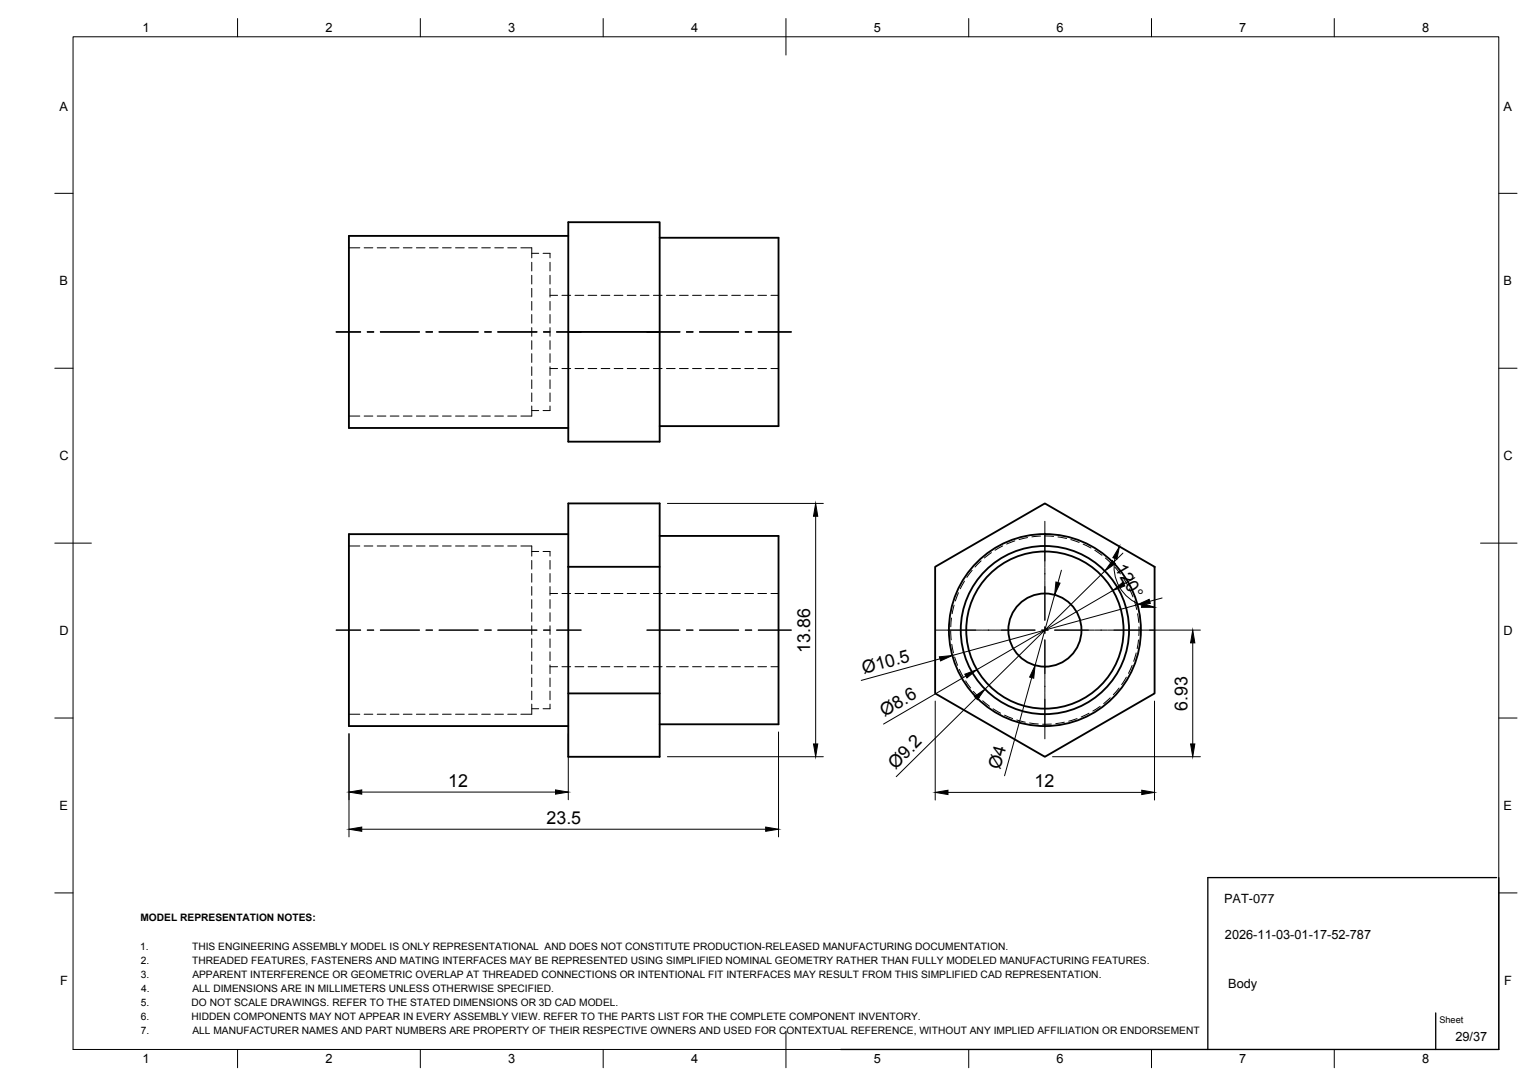
ISO-10303-21;
HEADER;
/* Generated by software containing ST-Developer
 * from STEP Tools, Inc. (www.steptools.com) 
 */

FILE_DESCRIPTION(
/* description */ ('Pallet stop with pneumatic fitting'),
/* implementation_level */ '2;1');

FILE_NAME(
/* name */ 'Body.step',
/* time_stamp */ '2026-10-27T10:51:41-07:00',
/* author */ (''),
/* organization */ (''),
/* preprocessor_version */ 'ST-DEVELOPER v20.2',
/* originating_system */ 'Autodesk Translation Framework v15.17.0.0',
/* authorisation */ '');

FILE_SCHEMA (('AUTOMOTIVE_DESIGN { 1 0 10303 214 3 1 1 }'));
ENDSEC;

DATA;
#10=MECHANICAL_DESIGN_GEOMETRIC_PRESENTATION_REPRESENTATION('',(#378),#10265);
#314=SHAPE_REPRESENTATION_RELATIONSHIP('SRR','None',#10429,#346);
#346=ADVANCED_BREP_SHAPE_REPRESENTATION('',(#409),#10253);
#378=STYLED_ITEM('',(#10634),#409);
#409=MANIFOLD_SOLID_BREP('Body1',#5067);
#516=FACE_BOUND('',#1349,.T.);
#517=FACE_BOUND('',#1351,.T.);
#518=FACE_BOUND('',#1353,.T.);
#519=FACE_BOUND('',#1361,.T.);
#520=FACE_BOUND('',#1364,.T.);
#521=FACE_BOUND('',#1368,.T.);
#660=PLANE('',#5834);
#661=PLANE('',#5836);
#662=PLANE('',#5838);
#663=PLANE('',#5840);
#664=PLANE('',#5841);
#665=PLANE('',#5842);
#666=PLANE('',#5843);
#667=PLANE('',#5844);
#668=PLANE('',#5845);
#669=PLANE('',#5846);
#670=PLANE('',#5850);
#671=PLANE('',#5855);
#936=FACE_OUTER_BOUND('',#1347,.T.);
#937=FACE_OUTER_BOUND('',#1348,.T.);
#938=FACE_OUTER_BOUND('',#1350,.T.);
#939=FACE_OUTER_BOUND('',#1352,.T.);
#940=FACE_OUTER_BOUND('',#1354,.T.);
#941=FACE_OUTER_BOUND('',#1355,.T.);
#942=FACE_OUTER_BOUND('',#1356,.T.);
#943=FACE_OUTER_BOUND('',#1357,.T.);
#944=FACE_OUTER_BOUND('',#1358,.T.);
#945=FACE_OUTER_BOUND('',#1359,.T.);
#946=FACE_OUTER_BOUND('',#1360,.T.);
#947=FACE_OUTER_BOUND('',#1362,.T.);
#948=FACE_OUTER_BOUND('',#1363,.T.);
#949=FACE_OUTER_BOUND('',#1365,.T.);
#950=FACE_OUTER_BOUND('',#1366,.T.);
#951=FACE_OUTER_BOUND('',#1367,.T.);
#952=FACE_OUTER_BOUND('',#1369,.T.);
#1347=EDGE_LOOP('',(#4160,#4161,#4162,#4163));
#1348=EDGE_LOOP('',(#4164));
#1349=EDGE_LOOP('',(#4165));
#1350=EDGE_LOOP('',(#4166,#4167,#4168,#4169,#4170,#4171));
#1351=EDGE_LOOP('',(#4172));
#1352=EDGE_LOOP('',(#4173,#4174,#4175,#4176,#4177,#4178));
#1353=EDGE_LOOP('',(#4179));
#1354=EDGE_LOOP('',(#4180,#4181,#4182,#4183));
#1355=EDGE_LOOP('',(#4184,#4185,#4186,#4187));
#1356=EDGE_LOOP('',(#4188,#4189,#4190,#4191));
#1357=EDGE_LOOP('',(#4192,#4193,#4194,#4195));
#1358=EDGE_LOOP('',(#4196,#4197,#4198,#4199));
#1359=EDGE_LOOP('',(#4200,#4201,#4202,#4203));
#1360=EDGE_LOOP('',(#4204));
#1361=EDGE_LOOP('',(#4205));
#1362=EDGE_LOOP('',(#4206,#4207,#4208,#4209));
#1363=EDGE_LOOP('',(#4210));
#1364=EDGE_LOOP('',(#4211));
#1365=EDGE_LOOP('',(#4212,#4213,#4214,#4215));
#1366=EDGE_LOOP('',(#4216,#4217,#4218,#4219));
#1367=EDGE_LOOP('',(#4220));
#1368=EDGE_LOOP('',(#4221));
#1369=EDGE_LOOP('',(#4222,#4223,#4224,#4225));
#1686=LINE('',#9545,#2021);
#1687=LINE('',#9553,#2022);
#1688=LINE('',#9555,#2023);
#1689=LINE('',#9557,#2024);
#1690=LINE('',#9559,#2025);
#1691=LINE('',#9561,#2026);
#1692=LINE('',#9562,#2027);
#1693=LINE('',#9568,#2028);
#1694=LINE('',#9570,#2029);
#1695=LINE('',#9572,#2030);
#1696=LINE('',#9574,#2031);
#1697=LINE('',#9576,#2032);
#1698=LINE('',#9577,#2033);
#1699=LINE('',#9581,#2034);
#1700=LINE('',#9582,#2035);
#1701=LINE('',#9584,#2036);
#1702=LINE('',#9586,#2037);
#1703=LINE('',#9588,#2038);
#1704=LINE('',#9590,#2039);
#1705=LINE('',#9597,#2040);
#1706=LINE('',#9603,#2041);
#1707=LINE('',#9607,#2042);
#1708=LINE('',#9612,#2043);
#2021=VECTOR('',#7087,0.43);
#2022=VECTOR('',#7096,1.);
#2023=VECTOR('',#7097,1.);
#2024=VECTOR('',#7098,1.);
#2025=VECTOR('',#7099,1.);
#2026=VECTOR('',#7100,1.);
#2027=VECTOR('',#7101,1.);
#2028=VECTOR('',#7106,1.);
#2029=VECTOR('',#7107,1.);
#2030=VECTOR('',#7108,1.);
#2031=VECTOR('',#7109,1.);
#2032=VECTOR('',#7110,1.);
#2033=VECTOR('',#7111,1.);
#2034=VECTOR('',#7116,1.);
#2035=VECTOR('',#7117,1.);
#2036=VECTOR('',#7120,1.);
#2037=VECTOR('',#7123,1.);
#2038=VECTOR('',#7126,1.);
#2039=VECTOR('',#7129,1.);
#2040=VECTOR('',#7138,0.46);
#2041=VECTOR('',#7147,0.525);
#2042=VECTOR('',#7152,0.515);
#2043=VECTOR('',#7159,0.2);
#2332=CIRCLE('',#5832,0.43);
#2333=CIRCLE('',#5833,0.43);
#2334=CIRCLE('',#5835,0.2);
#2335=CIRCLE('',#5837,0.525);
#2336=CIRCLE('',#5839,0.515);
#2337=CIRCLE('',#5847,0.46);
#2338=CIRCLE('',#5849,0.46);
#2339=CIRCLE('',#5851,0.525);
#2340=CIRCLE('',#5854,0.515);
#2341=CIRCLE('',#5856,0.2);
#2654=VERTEX_POINT('',#9542);
#2655=VERTEX_POINT('',#9544);
#2656=VERTEX_POINT('',#9548);
#2657=VERTEX_POINT('',#9551);
#2658=VERTEX_POINT('',#9552);
#2659=VERTEX_POINT('',#9554);
#2660=VERTEX_POINT('',#9556);
#2661=VERTEX_POINT('',#9558);
#2662=VERTEX_POINT('',#9560);
#2663=VERTEX_POINT('',#9563);
#2664=VERTEX_POINT('',#9566);
#2665=VERTEX_POINT('',#9567);
#2666=VERTEX_POINT('',#9569);
#2667=VERTEX_POINT('',#9571);
#2668=VERTEX_POINT('',#9573);
#2669=VERTEX_POINT('',#9575);
#2670=VERTEX_POINT('',#9578);
#2671=VERTEX_POINT('',#9593);
#2672=VERTEX_POINT('',#9596);
#2673=VERTEX_POINT('',#9600);
#2674=VERTEX_POINT('',#9605);
#2675=VERTEX_POINT('',#9609);
#3179=EDGE_CURVE('',#2654,#2654,#2332,.T.);
#3180=EDGE_CURVE('',#2654,#2655,#1686,.T.);
#3181=EDGE_CURVE('',#2655,#2655,#2333,.T.);
#3182=EDGE_CURVE('',#2656,#2656,#2334,.T.);
#3183=EDGE_CURVE('',#2657,#2658,#1687,.T.);
#3184=EDGE_CURVE('',#2658,#2659,#1688,.T.);
#3185=EDGE_CURVE('',#2659,#2660,#1689,.T.);
#3186=EDGE_CURVE('',#2660,#2661,#1690,.T.);
#3187=EDGE_CURVE('',#2661,#2662,#1691,.T.);
#3188=EDGE_CURVE('',#2662,#2657,#1692,.T.);
#3189=EDGE_CURVE('',#2663,#2663,#2335,.T.);
#3190=EDGE_CURVE('',#2664,#2665,#1693,.T.);
#3191=EDGE_CURVE('',#2666,#2664,#1694,.T.);
#3192=EDGE_CURVE('',#2667,#2666,#1695,.T.);
#3193=EDGE_CURVE('',#2668,#2667,#1696,.T.);
#3194=EDGE_CURVE('',#2669,#2668,#1697,.T.);
#3195=EDGE_CURVE('',#2665,#2669,#1698,.T.);
#3196=EDGE_CURVE('',#2670,#2670,#2336,.T.);
#3197=EDGE_CURVE('',#2664,#2657,#1699,.T.);
#3198=EDGE_CURVE('',#2666,#2662,#1700,.T.);
#3199=EDGE_CURVE('',#2667,#2661,#1701,.T.);
#3200=EDGE_CURVE('',#2668,#2660,#1702,.T.);
#3201=EDGE_CURVE('',#2669,#2659,#1703,.T.);
#3202=EDGE_CURVE('',#2665,#2658,#1704,.T.);
#3203=EDGE_CURVE('',#2671,#2671,#2337,.T.);
#3204=EDGE_CURVE('',#2671,#2672,#1705,.T.);
#3205=EDGE_CURVE('',#2672,#2672,#2338,.T.);
#3206=EDGE_CURVE('',#2673,#2673,#2339,.T.);
#3207=EDGE_CURVE('',#2663,#2673,#1706,.T.);
#3208=EDGE_CURVE('',#2674,#2674,#2340,.T.);
#3209=EDGE_CURVE('',#2674,#2670,#1707,.T.);
#3210=EDGE_CURVE('',#2675,#2675,#2341,.T.);
#3211=EDGE_CURVE('',#2675,#2656,#1708,.T.);
#4160=ORIENTED_EDGE('',*,*,#3179,.F.);
#4161=ORIENTED_EDGE('',*,*,#3180,.T.);
#4162=ORIENTED_EDGE('',*,*,#3181,.F.);
#4163=ORIENTED_EDGE('',*,*,#3180,.F.);
#4164=ORIENTED_EDGE('',*,*,#3179,.T.);
#4165=ORIENTED_EDGE('',*,*,#3182,.F.);
#4166=ORIENTED_EDGE('',*,*,#3183,.T.);
#4167=ORIENTED_EDGE('',*,*,#3184,.T.);
#4168=ORIENTED_EDGE('',*,*,#3185,.T.);
#4169=ORIENTED_EDGE('',*,*,#3186,.T.);
#4170=ORIENTED_EDGE('',*,*,#3187,.T.);
#4171=ORIENTED_EDGE('',*,*,#3188,.T.);
#4172=ORIENTED_EDGE('',*,*,#3189,.T.);
#4173=ORIENTED_EDGE('',*,*,#3190,.F.);
#4174=ORIENTED_EDGE('',*,*,#3191,.F.);
#4175=ORIENTED_EDGE('',*,*,#3192,.F.);
#4176=ORIENTED_EDGE('',*,*,#3193,.F.);
#4177=ORIENTED_EDGE('',*,*,#3194,.F.);
#4178=ORIENTED_EDGE('',*,*,#3195,.F.);
#4179=ORIENTED_EDGE('',*,*,#3196,.F.);
#4180=ORIENTED_EDGE('',*,*,#3191,.T.);
#4181=ORIENTED_EDGE('',*,*,#3197,.T.);
#4182=ORIENTED_EDGE('',*,*,#3188,.F.);
#4183=ORIENTED_EDGE('',*,*,#3198,.F.);
#4184=ORIENTED_EDGE('',*,*,#3192,.T.);
#4185=ORIENTED_EDGE('',*,*,#3198,.T.);
#4186=ORIENTED_EDGE('',*,*,#3187,.F.);
#4187=ORIENTED_EDGE('',*,*,#3199,.F.);
#4188=ORIENTED_EDGE('',*,*,#3193,.T.);
#4189=ORIENTED_EDGE('',*,*,#3199,.T.);
#4190=ORIENTED_EDGE('',*,*,#3186,.F.);
#4191=ORIENTED_EDGE('',*,*,#3200,.F.);
#4192=ORIENTED_EDGE('',*,*,#3194,.T.);
#4193=ORIENTED_EDGE('',*,*,#3200,.T.);
#4194=ORIENTED_EDGE('',*,*,#3185,.F.);
#4195=ORIENTED_EDGE('',*,*,#3201,.F.);
#4196=ORIENTED_EDGE('',*,*,#3195,.T.);
#4197=ORIENTED_EDGE('',*,*,#3201,.T.);
#4198=ORIENTED_EDGE('',*,*,#3184,.F.);
#4199=ORIENTED_EDGE('',*,*,#3202,.F.);
#4200=ORIENTED_EDGE('',*,*,#3190,.T.);
#4201=ORIENTED_EDGE('',*,*,#3202,.T.);
#4202=ORIENTED_EDGE('',*,*,#3183,.F.);
#4203=ORIENTED_EDGE('',*,*,#3197,.F.);
#4204=ORIENTED_EDGE('',*,*,#3203,.F.);
#4205=ORIENTED_EDGE('',*,*,#3181,.T.);
#4206=ORIENTED_EDGE('',*,*,#3203,.T.);
#4207=ORIENTED_EDGE('',*,*,#3204,.T.);
#4208=ORIENTED_EDGE('',*,*,#3205,.F.);
#4209=ORIENTED_EDGE('',*,*,#3204,.F.);
#4210=ORIENTED_EDGE('',*,*,#3206,.F.);
#4211=ORIENTED_EDGE('',*,*,#3205,.T.);
#4212=ORIENTED_EDGE('',*,*,#3189,.F.);
#4213=ORIENTED_EDGE('',*,*,#3207,.T.);
#4214=ORIENTED_EDGE('',*,*,#3206,.T.);
#4215=ORIENTED_EDGE('',*,*,#3207,.F.);
#4216=ORIENTED_EDGE('',*,*,#3208,.F.);
#4217=ORIENTED_EDGE('',*,*,#3209,.T.);
#4218=ORIENTED_EDGE('',*,*,#3196,.T.);
#4219=ORIENTED_EDGE('',*,*,#3209,.F.);
#4220=ORIENTED_EDGE('',*,*,#3208,.T.);
#4221=ORIENTED_EDGE('',*,*,#3210,.F.);
#4222=ORIENTED_EDGE('',*,*,#3210,.T.);
#4223=ORIENTED_EDGE('',*,*,#3211,.T.);
#4224=ORIENTED_EDGE('',*,*,#3182,.T.);
#4225=ORIENTED_EDGE('',*,*,#3211,.F.);
#4702=CYLINDRICAL_SURFACE('',#5831,0.43);
#4703=CYLINDRICAL_SURFACE('',#5848,0.46);
#4704=CYLINDRICAL_SURFACE('',#5852,0.525);
#4705=CYLINDRICAL_SURFACE('',#5853,0.515);
#4706=CYLINDRICAL_SURFACE('',#5857,0.2);
#4931=ADVANCED_FACE('',(#936),#4702,.F.);
#4932=ADVANCED_FACE('',(#937,#516),#660,.T.);
#4933=ADVANCED_FACE('',(#938,#517),#661,.T.);
#4934=ADVANCED_FACE('',(#939,#518),#662,.F.);
#4935=ADVANCED_FACE('',(#940),#663,.T.);
#4936=ADVANCED_FACE('',(#941),#664,.T.);
#4937=ADVANCED_FACE('',(#942),#665,.T.);
#4938=ADVANCED_FACE('',(#943),#666,.T.);
#4939=ADVANCED_FACE('',(#944),#667,.T.);
#4940=ADVANCED_FACE('',(#945),#668,.T.);
#4941=ADVANCED_FACE('',(#946,#519),#669,.T.);
#4942=ADVANCED_FACE('',(#947),#4703,.F.);
#4943=ADVANCED_FACE('',(#948,#520),#670,.T.);
#4944=ADVANCED_FACE('',(#949),#4704,.T.);
#4945=ADVANCED_FACE('',(#950),#4705,.T.);
#4946=ADVANCED_FACE('',(#951,#521),#671,.T.);
#4947=ADVANCED_FACE('',(#952),#4706,.F.);
#5067=CLOSED_SHELL('',(#4931,#4932,#4933,#4934,#4935,#4936,#4937,#4938,
#4939,#4940,#4941,#4942,#4943,#4944,#4945,#4946,#4947));
#5830=AXIS2_PLACEMENT_3D('',#9540,#7081,#7082);
#5831=AXIS2_PLACEMENT_3D('',#9541,#7083,#7084);
#5832=AXIS2_PLACEMENT_3D('',#9543,#7085,#7086);
#5833=AXIS2_PLACEMENT_3D('',#9546,#7088,#7089);
#5834=AXIS2_PLACEMENT_3D('',#9547,#7090,#7091);
#5835=AXIS2_PLACEMENT_3D('',#9549,#7092,#7093);
#5836=AXIS2_PLACEMENT_3D('',#9550,#7094,#7095);
#5837=AXIS2_PLACEMENT_3D('',#9564,#7102,#7103);
#5838=AXIS2_PLACEMENT_3D('',#9565,#7104,#7105);
#5839=AXIS2_PLACEMENT_3D('',#9579,#7112,#7113);
#5840=AXIS2_PLACEMENT_3D('',#9580,#7114,#7115);
#5841=AXIS2_PLACEMENT_3D('',#9583,#7118,#7119);
#5842=AXIS2_PLACEMENT_3D('',#9585,#7121,#7122);
#5843=AXIS2_PLACEMENT_3D('',#9587,#7124,#7125);
#5844=AXIS2_PLACEMENT_3D('',#9589,#7127,#7128);
#5845=AXIS2_PLACEMENT_3D('',#9591,#7130,#7131);
#5846=AXIS2_PLACEMENT_3D('',#9592,#7132,#7133);
#5847=AXIS2_PLACEMENT_3D('',#9594,#7134,#7135);
#5848=AXIS2_PLACEMENT_3D('',#9595,#7136,#7137);
#5849=AXIS2_PLACEMENT_3D('',#9598,#7139,#7140);
#5850=AXIS2_PLACEMENT_3D('',#9599,#7141,#7142);
#5851=AXIS2_PLACEMENT_3D('',#9601,#7143,#7144);
#5852=AXIS2_PLACEMENT_3D('',#9602,#7145,#7146);
#5853=AXIS2_PLACEMENT_3D('',#9604,#7148,#7149);
#5854=AXIS2_PLACEMENT_3D('',#9606,#7150,#7151);
#5855=AXIS2_PLACEMENT_3D('',#9608,#7153,#7154);
#5856=AXIS2_PLACEMENT_3D('',#9610,#7155,#7156);
#5857=AXIS2_PLACEMENT_3D('',#9611,#7157,#7158);
#7081=DIRECTION('axis',(0.,0.,1.));
#7082=DIRECTION('refdir',(1.,0.,0.));
#7083=DIRECTION('center_axis',(0.,1.,0.));
#7084=DIRECTION('ref_axis',(1.,0.,0.));
#7085=DIRECTION('center_axis',(0.,1.,0.));
#7086=DIRECTION('ref_axis',(1.,0.,0.));
#7087=DIRECTION('',(0.,1.,0.));
#7088=DIRECTION('center_axis',(0.,-1.,0.));
#7089=DIRECTION('ref_axis',(1.,0.,0.));
#7090=DIRECTION('center_axis',(0.,1.,0.));
#7091=DIRECTION('ref_axis',(1.,0.,0.));
#7092=DIRECTION('center_axis',(0.,1.,0.));
#7093=DIRECTION('ref_axis',(1.,0.,0.));
#7094=DIRECTION('center_axis',(0.,1.,0.));
#7095=DIRECTION('ref_axis',(1.,0.,0.));
#7096=DIRECTION('',(0.5,0.,-0.866025403784439));
#7097=DIRECTION('',(-0.5,0.,-0.866025403784439));
#7098=DIRECTION('',(-1.,0.,-1.60246890531964E-16));
#7099=DIRECTION('',(-0.5,0.,0.866025403784439));
#7100=DIRECTION('',(0.5,0.,0.866025403784439));
#7101=DIRECTION('',(1.,0.,1.60246890531964E-16));
#7102=DIRECTION('center_axis',(0.,-1.,0.));
#7103=DIRECTION('ref_axis',(1.,0.,0.));
#7104=DIRECTION('center_axis',(0.,1.,0.));
#7105=DIRECTION('ref_axis',(1.,0.,0.));
#7106=DIRECTION('',(0.5,0.,-0.866025403784439));
#7107=DIRECTION('',(1.,0.,1.60246890531964E-16));
#7108=DIRECTION('',(0.5,0.,0.866025403784439));
#7109=DIRECTION('',(-0.5,0.,0.866025403784439));
#7110=DIRECTION('',(-1.,0.,-1.60246890531964E-16));
#7111=DIRECTION('',(-0.5,0.,-0.866025403784439));
#7112=DIRECTION('center_axis',(0.,-1.,0.));
#7113=DIRECTION('ref_axis',(1.,0.,0.));
#7114=DIRECTION('center_axis',(-1.60246890531964E-16,0.,1.));
#7115=DIRECTION('ref_axis',(1.,0.,1.60246890531964E-16));
#7116=DIRECTION('',(0.,1.,0.));
#7117=DIRECTION('',(0.,1.,0.));
#7118=DIRECTION('center_axis',(-0.866025403784439,0.,0.5));
#7119=DIRECTION('ref_axis',(0.5,0.,0.866025403784439));
#7120=DIRECTION('',(0.,1.,0.));
#7121=DIRECTION('center_axis',(-0.866025403784439,0.,-0.5));
#7122=DIRECTION('ref_axis',(-0.5,0.,0.866025403784439));
#7123=DIRECTION('',(0.,1.,0.));
#7124=DIRECTION('center_axis',(1.60246890531964E-16,0.,-1.));
#7125=DIRECTION('ref_axis',(-1.,0.,-1.60246890531964E-16));
#7126=DIRECTION('',(0.,1.,0.));
#7127=DIRECTION('center_axis',(0.866025403784439,0.,-0.5));
#7128=DIRECTION('ref_axis',(-0.5,0.,-0.866025403784439));
#7129=DIRECTION('',(0.,1.,0.));
#7130=DIRECTION('center_axis',(0.866025403784439,0.,0.5));
#7131=DIRECTION('ref_axis',(0.5,0.,-0.866025403784439));
#7132=DIRECTION('center_axis',(0.,1.,0.));
#7133=DIRECTION('ref_axis',(0.,0.,1.));
#7134=DIRECTION('center_axis',(0.,-1.,0.));
#7135=DIRECTION('ref_axis',(1.,0.,0.));
#7136=DIRECTION('center_axis',(0.,-1.,0.));
#7137=DIRECTION('ref_axis',(1.,0.,0.));
#7138=DIRECTION('',(0.,1.,0.));
#7139=DIRECTION('center_axis',(0.,-1.,0.));
#7140=DIRECTION('ref_axis',(1.,0.,0.));
#7141=DIRECTION('center_axis',(0.,1.,0.));
#7142=DIRECTION('ref_axis',(0.,0.,1.));
#7143=DIRECTION('center_axis',(0.,-1.,0.));
#7144=DIRECTION('ref_axis',(1.,0.,0.));
#7145=DIRECTION('center_axis',(0.,-1.,0.));
#7146=DIRECTION('ref_axis',(1.,0.,0.));
#7147=DIRECTION('',(0.,1.,0.));
#7148=DIRECTION('center_axis',(0.,-1.,0.));
#7149=DIRECTION('ref_axis',(1.,0.,0.));
#7150=DIRECTION('center_axis',(0.,-1.,0.));
#7151=DIRECTION('ref_axis',(1.,0.,0.));
#7152=DIRECTION('',(0.,1.,0.));
#7153=DIRECTION('center_axis',(0.,-1.,0.));
#7154=DIRECTION('ref_axis',(0.,0.,-1.));
#7155=DIRECTION('center_axis',(0.,-1.,0.));
#7156=DIRECTION('ref_axis',(1.,0.,0.));
#7157=DIRECTION('center_axis',(0.,-1.,0.));
#7158=DIRECTION('ref_axis',(1.,0.,0.));
#7159=DIRECTION('',(0.,1.,0.));
#9540=CARTESIAN_POINT('',(0.,0.,0.));
#9541=CARTESIAN_POINT('Origin',(0.,0.6,0.));
#9542=CARTESIAN_POINT('',(-0.43,0.6,5.26598123633362E-17));
#9543=CARTESIAN_POINT('Origin',(0.,0.6,0.));
#9544=CARTESIAN_POINT('',(-0.43,0.7,-5.26598123633362E-17));
#9545=CARTESIAN_POINT('',(-0.43,0.6,5.26598123633362E-17));
#9546=CARTESIAN_POINT('Origin',(0.,0.7,0.));
#9547=CARTESIAN_POINT('Origin',(0.,0.6,0.));
#9548=CARTESIAN_POINT('',(-0.2,0.6,2.44929359829471E-17));
#9549=CARTESIAN_POINT('Origin',(0.,0.6,0.));
#9550=CARTESIAN_POINT('Origin',(0.,0.5,-1.11022302462516E-16));
#9551=CARTESIAN_POINT('',(0.346410161513776,0.5,0.6));
#9552=CARTESIAN_POINT('',(0.692820323027551,0.5,0.));
#9553=CARTESIAN_POINT('',(0.346410161513776,0.5,0.6));
#9554=CARTESIAN_POINT('',(0.346410161513776,0.5,-0.6));
#9555=CARTESIAN_POINT('',(0.692820323027551,0.5,0.));
#9556=CARTESIAN_POINT('',(-0.346410161513775,0.5,-0.6));
#9557=CARTESIAN_POINT('',(0.346410161513776,0.5,-0.6));
#9558=CARTESIAN_POINT('',(-0.692820323027551,0.5,-8.48460190979926E-17));
#9559=CARTESIAN_POINT('',(-0.346410161513775,0.5,-0.6));
#9560=CARTESIAN_POINT('',(-0.346410161513776,0.5,0.6));
#9561=CARTESIAN_POINT('',(-0.692820323027551,0.5,-8.48460190979926E-17));
#9562=CARTESIAN_POINT('',(-0.346410161513776,0.5,0.6));
#9563=CARTESIAN_POINT('',(-0.525,0.5,-6.4293956955236E-17));
#9564=CARTESIAN_POINT('Origin',(0.,0.5,0.));
#9565=CARTESIAN_POINT('Origin',(0.,0.,-1.11022302462516E-16));
#9566=CARTESIAN_POINT('',(0.346410161513776,0.,0.6));
#9567=CARTESIAN_POINT('',(0.692820323027551,0.,0.));
#9568=CARTESIAN_POINT('',(0.346410161513776,0.,0.6));
#9569=CARTESIAN_POINT('',(-0.346410161513776,0.,0.6));
#9570=CARTESIAN_POINT('',(-0.346410161513776,0.,0.6));
#9571=CARTESIAN_POINT('',(-0.692820323027551,0.,-8.48460190979926E-17));
#9572=CARTESIAN_POINT('',(-0.692820323027551,0.,-8.48460190979926E-17));
#9573=CARTESIAN_POINT('',(-0.346410161513775,0.,-0.6));
#9574=CARTESIAN_POINT('',(-0.346410161513775,0.,-0.6));
#9575=CARTESIAN_POINT('',(0.346410161513776,0.,-0.6));
#9576=CARTESIAN_POINT('',(0.346410161513776,0.,-0.6));
#9577=CARTESIAN_POINT('',(0.692820323027551,0.,0.));
#9578=CARTESIAN_POINT('',(-0.515,0.,-6.30693101560887E-17));
#9579=CARTESIAN_POINT('Origin',(0.,0.,0.));
#9580=CARTESIAN_POINT('Origin',(-0.346410161513776,0.,0.6));
#9581=CARTESIAN_POINT('',(0.346410161513776,0.,0.6));
#9582=CARTESIAN_POINT('',(-0.346410161513776,0.,0.6));
#9583=CARTESIAN_POINT('Origin',(-0.692820323027551,0.,-8.48460190979926E-17));
#9584=CARTESIAN_POINT('',(-0.692820323027551,0.,-8.48460190979926E-17));
#9585=CARTESIAN_POINT('Origin',(-0.346410161513775,0.,-0.6));
#9586=CARTESIAN_POINT('',(-0.346410161513775,0.,-0.6));
#9587=CARTESIAN_POINT('Origin',(0.346410161513776,0.,-0.6));
#9588=CARTESIAN_POINT('',(0.346410161513776,0.,-0.6));
#9589=CARTESIAN_POINT('Origin',(0.692820323027551,0.,0.));
#9590=CARTESIAN_POINT('',(0.692820323027551,0.,0.));
#9591=CARTESIAN_POINT('Origin',(0.346410161513776,0.,0.6));
#9592=CARTESIAN_POINT('Origin',(0.46,0.7,0.));
#9593=CARTESIAN_POINT('',(-0.46,0.7,-5.63337527607782E-17));
#9594=CARTESIAN_POINT('Origin',(0.,0.7,0.));
#9595=CARTESIAN_POINT('Origin',(0.,1.2,0.));
#9596=CARTESIAN_POINT('',(-0.46,1.7,-5.63337527607782E-17));
#9597=CARTESIAN_POINT('',(-0.46,1.2,-5.63337527607782E-17));
#9598=CARTESIAN_POINT('Origin',(0.,1.7,0.));
#9599=CARTESIAN_POINT('Origin',(0.525,1.7,0.));
#9600=CARTESIAN_POINT('',(-0.525,1.7,-6.4293956955236E-17));
#9601=CARTESIAN_POINT('Origin',(0.,1.7,0.));
#9602=CARTESIAN_POINT('Origin',(0.,1.1,0.));
#9603=CARTESIAN_POINT('',(-0.525,1.1,-6.4293956955236E-17));
#9604=CARTESIAN_POINT('Origin',(0.,-0.325,0.));
#9605=CARTESIAN_POINT('',(-0.515,-0.65,-6.30693101560887E-17));
#9606=CARTESIAN_POINT('Origin',(0.,-0.65,0.));
#9607=CARTESIAN_POINT('',(-0.515,-0.325,-6.30693101560887E-17));
#9608=CARTESIAN_POINT('Origin',(0.2,-0.65,0.));
#9609=CARTESIAN_POINT('',(-0.2,-0.65,-2.44929359829471E-17));
#9610=CARTESIAN_POINT('Origin',(0.,-0.65,0.));
#9611=CARTESIAN_POINT('Origin',(0.,0.0249999999999999,0.));
#9612=CARTESIAN_POINT('',(-0.2,0.0249999999999999,-2.44929359829471E-17));
#10215=UNCERTAINTY_MEASURE_WITH_UNIT(LENGTH_MEASURE(0.001),#10266,
'DISTANCE_ACCURACY_VALUE',
'Maximum model space distance between geometric entities at asserted c
onnectivities');
#10227=UNCERTAINTY_MEASURE_WITH_UNIT(LENGTH_MEASURE(0.001),#10266,
'DISTANCE_ACCURACY_VALUE',
'Maximum model space distance between geometric entities at asserted c
onnectivities');
#10253=(
GEOMETRIC_REPRESENTATION_CONTEXT(3)
GLOBAL_UNCERTAINTY_ASSIGNED_CONTEXT((#10215))
GLOBAL_UNIT_ASSIGNED_CONTEXT((#10266,#10268,#10269))
REPRESENTATION_CONTEXT('','3D')
);
#10265=(
GEOMETRIC_REPRESENTATION_CONTEXT(3)
GLOBAL_UNCERTAINTY_ASSIGNED_CONTEXT((#10227))
GLOBAL_UNIT_ASSIGNED_CONTEXT((#10266,#10268,#10269))
REPRESENTATION_CONTEXT('','3D')
);
#10266=(
LENGTH_UNIT()
NAMED_UNIT(*)
SI_UNIT(.CENTI.,.METRE.)
);
#10268=(
NAMED_UNIT(*)
PLANE_ANGLE_UNIT()
SI_UNIT($,.RADIAN.)
);
#10269=(
NAMED_UNIT(*)
SI_UNIT($,.STERADIAN.)
SOLID_ANGLE_UNIT()
);
#10295=SHAPE_DEFINITION_REPRESENTATION(#10334,#10429);
#10334=PRODUCT_DEFINITION_SHAPE('',$,#10467);
#10429=SHAPE_REPRESENTATION('',(#5830),#10253);
#10441=PRODUCT_DEFINITION_CONTEXT('part definition',#10554,'design');
#10467=PRODUCT_DEFINITION('Body','Body',#10504,#10441);
#10504=PRODUCT_DEFINITION_FORMATION('',$,#10581);
#10554=APPLICATION_CONTEXT(
'Core Data for Automotive Mechanical Design Process');
#10555=PRODUCT_CONTEXT('part definition',#10554,'mechanical');
#10581=PRODUCT('Body','Body','Body',(#10555));
#10628=COLOUR_RGB('Dark Blue',0.08,0.2,0.34);
#10629=FILL_AREA_STYLE_COLOUR('',#10628);
#10630=FILL_AREA_STYLE('',(#10629));
#10631=SURFACE_STYLE_FILL_AREA(#10630);
#10632=SURFACE_SIDE_STYLE('',(#10631));
#10633=SURFACE_STYLE_USAGE(.BOTH.,#10632);
#10634=PRESENTATION_STYLE_ASSIGNMENT((#10633));
ENDSEC;
END-ISO-10303-21;
